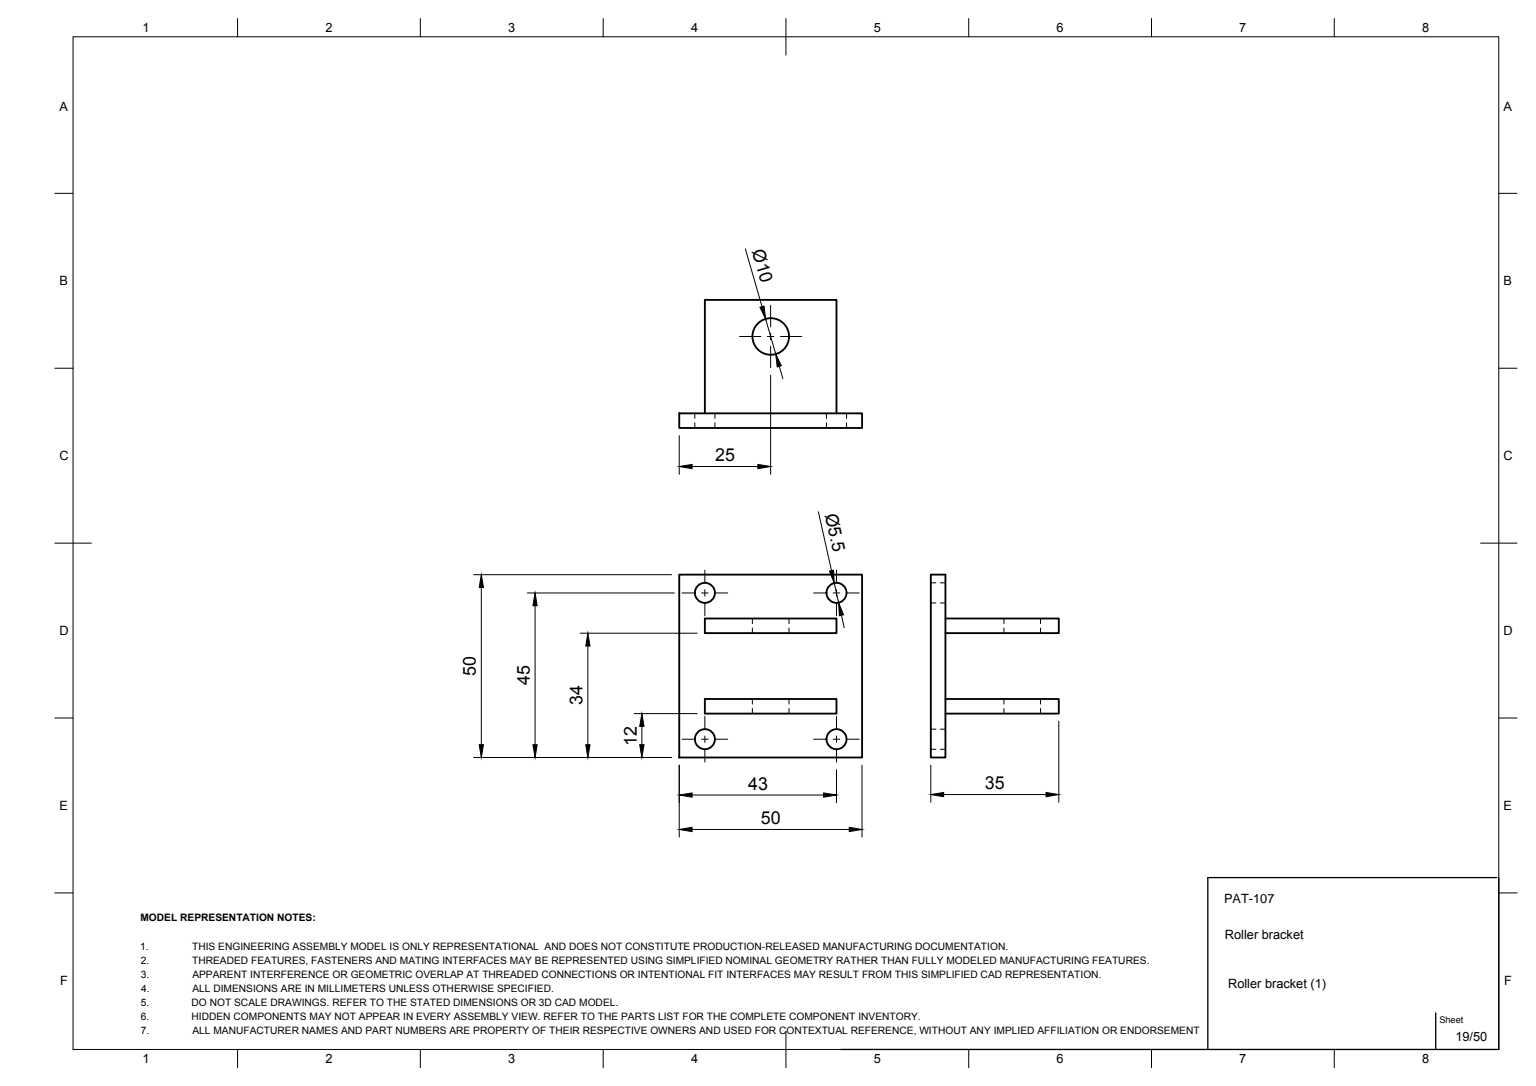
ISO-10303-21;
HEADER;
/* Generated by software containing ST-Developer
 * from STEP Tools, Inc. (www.steptools.com) 
 */

FILE_DESCRIPTION(
/* description */ ('Turntable on roller ring'),
/* implementation_level */ '2;1');

FILE_NAME(
/* name */ 'Roller bracket.step',
/* time_stamp */ '2026-10-28T03:23:59-07:00',
/* author */ (''),
/* organization */ (''),
/* preprocessor_version */ 'ST-DEVELOPER v20.2',
/* originating_system */ 'Autodesk Translation Framework v15.17.0.0',
/* authorisation */ '');

FILE_SCHEMA (('AUTOMOTIVE_DESIGN { 1 0 10303 214 3 1 1 }'));
ENDSEC;

DATA;
#10=MECHANICAL_DESIGN_GEOMETRIC_PRESENTATION_REPRESENTATION('',(#642),#16281);
#523=SHAPE_REPRESENTATION_RELATIONSHIP('SRR','None',#16540,#578);
#578=ADVANCED_BREP_SHAPE_REPRESENTATION('',(#712),#16234);
#642=STYLED_ITEM('',(#16911),#712);
#712=MANIFOLD_SOLID_BREP('Body1',#8385);
#867=FACE_BOUND('',#2085,.T.);
#868=FACE_BOUND('',#2087,.T.);
#869=FACE_BOUND('',#2092,.T.);
#870=FACE_BOUND('',#2094,.T.);
#871=FACE_BOUND('',#2100,.T.);
#872=FACE_BOUND('',#2101,.T.);
#873=FACE_BOUND('',#2102,.T.);
#874=FACE_BOUND('',#2103,.T.);
#875=FACE_BOUND('',#2104,.T.);
#876=FACE_BOUND('',#2105,.T.);
#877=FACE_BOUND('',#2107,.T.);
#878=FACE_BOUND('',#2108,.T.);
#879=FACE_BOUND('',#2109,.T.);
#880=FACE_BOUND('',#2110,.T.);
#1083=PLANE('',#9552);
#1084=PLANE('',#9553);
#1085=PLANE('',#9554);
#1086=PLANE('',#9555);
#1087=PLANE('',#9556);
#1088=PLANE('',#9557);
#1089=PLANE('',#9558);
#1090=PLANE('',#9559);
#1091=PLANE('',#9560);
#1092=PLANE('',#9561);
#1093=PLANE('',#9562);
#1094=PLANE('',#9563);
#1095=PLANE('',#9564);
#1096=PLANE('',#9565);
#1097=PLANE('',#9566);
#1098=PLANE('',#9567);
#1460=FACE_OUTER_BOUND('',#2075,.T.);
#1461=FACE_OUTER_BOUND('',#2076,.T.);
#1462=FACE_OUTER_BOUND('',#2077,.T.);
#1463=FACE_OUTER_BOUND('',#2078,.T.);
#1464=FACE_OUTER_BOUND('',#2079,.T.);
#1465=FACE_OUTER_BOUND('',#2080,.T.);
#1466=FACE_OUTER_BOUND('',#2081,.T.);
#1467=FACE_OUTER_BOUND('',#2082,.T.);
#1468=FACE_OUTER_BOUND('',#2083,.T.);
#1469=FACE_OUTER_BOUND('',#2084,.T.);
#1470=FACE_OUTER_BOUND('',#2086,.T.);
#1471=FACE_OUTER_BOUND('',#2088,.T.);
#1472=FACE_OUTER_BOUND('',#2089,.T.);
#1473=FACE_OUTER_BOUND('',#2090,.T.);
#1474=FACE_OUTER_BOUND('',#2091,.T.);
#1475=FACE_OUTER_BOUND('',#2093,.T.);
#1476=FACE_OUTER_BOUND('',#2095,.T.);
#1477=FACE_OUTER_BOUND('',#2096,.T.);
#1478=FACE_OUTER_BOUND('',#2097,.T.);
#1479=FACE_OUTER_BOUND('',#2098,.T.);
#1480=FACE_OUTER_BOUND('',#2099,.T.);
#1481=FACE_OUTER_BOUND('',#2106,.T.);
#2075=EDGE_LOOP('',(#6545,#6546,#6547,#6548));
#2076=EDGE_LOOP('',(#6549,#6550,#6551,#6552));
#2077=EDGE_LOOP('',(#6553,#6554,#6555,#6556));
#2078=EDGE_LOOP('',(#6557,#6558,#6559,#6560));
#2079=EDGE_LOOP('',(#6561,#6562,#6563,#6564));
#2080=EDGE_LOOP('',(#6565,#6566,#6567,#6568));
#2081=EDGE_LOOP('',(#6569,#6570,#6571,#6572));
#2082=EDGE_LOOP('',(#6573,#6574,#6575,#6576));
#2083=EDGE_LOOP('',(#6577,#6578,#6579,#6580));
#2084=EDGE_LOOP('',(#6581,#6582,#6583,#6584));
#2085=EDGE_LOOP('',(#6585));
#2086=EDGE_LOOP('',(#6586,#6587,#6588,#6589));
#2087=EDGE_LOOP('',(#6590));
#2088=EDGE_LOOP('',(#6591,#6592,#6593,#6594));
#2089=EDGE_LOOP('',(#6595,#6596,#6597,#6598));
#2090=EDGE_LOOP('',(#6599,#6600,#6601,#6602));
#2091=EDGE_LOOP('',(#6603,#6604,#6605,#6606));
#2092=EDGE_LOOP('',(#6607));
#2093=EDGE_LOOP('',(#6608,#6609,#6610,#6611));
#2094=EDGE_LOOP('',(#6612));
#2095=EDGE_LOOP('',(#6613,#6614,#6615,#6616));
#2096=EDGE_LOOP('',(#6617,#6618,#6619,#6620));
#2097=EDGE_LOOP('',(#6621,#6622,#6623,#6624));
#2098=EDGE_LOOP('',(#6625,#6626,#6627,#6628));
#2099=EDGE_LOOP('',(#6629,#6630,#6631,#6632));
#2100=EDGE_LOOP('',(#6633,#6634,#6635,#6636));
#2101=EDGE_LOOP('',(#6637,#6638,#6639,#6640));
#2102=EDGE_LOOP('',(#6641));
#2103=EDGE_LOOP('',(#6642));
#2104=EDGE_LOOP('',(#6643));
#2105=EDGE_LOOP('',(#6644));
#2106=EDGE_LOOP('',(#6645,#6646,#6647,#6648));
#2107=EDGE_LOOP('',(#6649));
#2108=EDGE_LOOP('',(#6650));
#2109=EDGE_LOOP('',(#6651));
#2110=EDGE_LOOP('',(#6652));
#2686=LINE('',#14454,#3169);
#2687=LINE('',#14460,#3170);
#2688=LINE('',#14466,#3171);
#2689=LINE('',#14472,#3172);
#2690=LINE('',#14478,#3173);
#2691=LINE('',#14484,#3174);
#2692=LINE('',#14489,#3175);
#2693=LINE('',#14491,#3176);
#2694=LINE('',#14493,#3177);
#2695=LINE('',#14494,#3178);
#2696=LINE('',#14498,#3179);
#2697=LINE('',#14500,#3180);
#2698=LINE('',#14502,#3181);
#2699=LINE('',#14503,#3182);
#2700=LINE('',#14505,#3183);
#2701=LINE('',#14506,#3184);
#2702=LINE('',#14508,#3185);
#2703=LINE('',#14510,#3186);
#2704=LINE('',#14514,#3187);
#2705=LINE('',#14516,#3188);
#2706=LINE('',#14518,#3189);
#2707=LINE('',#14519,#3190);
#2708=LINE('',#14523,#3191);
#2709=LINE('',#14525,#3192);
#2710=LINE('',#14527,#3193);
#2711=LINE('',#14528,#3194);
#2712=LINE('',#14530,#3195);
#2713=LINE('',#14531,#3196);
#2714=LINE('',#14533,#3197);
#2715=LINE('',#14535,#3198);
#2716=LINE('',#14539,#3199);
#2717=LINE('',#14541,#3200);
#2718=LINE('',#14543,#3201);
#2719=LINE('',#14544,#3202);
#2720=LINE('',#14547,#3203);
#2721=LINE('',#14549,#3204);
#2722=LINE('',#14550,#3205);
#2723=LINE('',#14553,#3206);
#2724=LINE('',#14555,#3207);
#2725=LINE('',#14556,#3208);
#2726=LINE('',#14558,#3209);
#2727=LINE('',#14559,#3210);
#3169=VECTOR('',#11385,0.275);
#3170=VECTOR('',#11392,0.275);
#3171=VECTOR('',#11399,0.275);
#3172=VECTOR('',#11406,0.275);
#3173=VECTOR('',#11413,0.5);
#3174=VECTOR('',#11420,0.5);
#3175=VECTOR('',#11425,1.);
#3176=VECTOR('',#11426,1.);
#3177=VECTOR('',#11427,1.);
#3178=VECTOR('',#11428,1.);
#3179=VECTOR('',#11431,1.);
#3180=VECTOR('',#11432,1.);
#3181=VECTOR('',#11433,1.);
#3182=VECTOR('',#11434,1.);
#3183=VECTOR('',#11437,1.);
#3184=VECTOR('',#11438,1.);
#3185=VECTOR('',#11441,1.);
#3186=VECTOR('',#11444,1.);
#3187=VECTOR('',#11447,1.);
#3188=VECTOR('',#11448,1.);
#3189=VECTOR('',#11449,1.);
#3190=VECTOR('',#11450,1.);
#3191=VECTOR('',#11453,1.);
#3192=VECTOR('',#11454,1.);
#3193=VECTOR('',#11455,1.);
#3194=VECTOR('',#11456,1.);
#3195=VECTOR('',#11459,1.);
#3196=VECTOR('',#11460,1.);
#3197=VECTOR('',#11463,1.);
#3198=VECTOR('',#11466,1.);
#3199=VECTOR('',#11469,1.);
#3200=VECTOR('',#11470,1.);
#3201=VECTOR('',#11471,1.);
#3202=VECTOR('',#11472,1.);
#3203=VECTOR('',#11475,1.);
#3204=VECTOR('',#11476,1.);
#3205=VECTOR('',#11477,1.);
#3206=VECTOR('',#11480,1.);
#3207=VECTOR('',#11481,1.);
#3208=VECTOR('',#11482,1.);
#3209=VECTOR('',#11485,1.);
#3210=VECTOR('',#11486,1.);
#3695=CIRCLE('',#9535,0.275);
#3696=CIRCLE('',#9536,0.275);
#3697=CIRCLE('',#9538,0.275);
#3698=CIRCLE('',#9539,0.275);
#3699=CIRCLE('',#9541,0.275);
#3700=CIRCLE('',#9542,0.275);
#3701=CIRCLE('',#9544,0.275);
#3702=CIRCLE('',#9545,0.275);
#3703=CIRCLE('',#9547,0.5);
#3704=CIRCLE('',#9548,0.5);
#3705=CIRCLE('',#9550,0.5);
#3706=CIRCLE('',#9551,0.5);
#4251=VERTEX_POINT('',#14451);
#4252=VERTEX_POINT('',#14453);
#4253=VERTEX_POINT('',#14457);
#4254=VERTEX_POINT('',#14459);
#4255=VERTEX_POINT('',#14463);
#4256=VERTEX_POINT('',#14465);
#4257=VERTEX_POINT('',#14469);
#4258=VERTEX_POINT('',#14471);
#4259=VERTEX_POINT('',#14475);
#4260=VERTEX_POINT('',#14477);
#4261=VERTEX_POINT('',#14481);
#4262=VERTEX_POINT('',#14483);
#4263=VERTEX_POINT('',#14487);
#4264=VERTEX_POINT('',#14488);
#4265=VERTEX_POINT('',#14490);
#4266=VERTEX_POINT('',#14492);
#4267=VERTEX_POINT('',#14496);
#4268=VERTEX_POINT('',#14497);
#4269=VERTEX_POINT('',#14499);
#4270=VERTEX_POINT('',#14501);
#4271=VERTEX_POINT('',#14512);
#4272=VERTEX_POINT('',#14513);
#4273=VERTEX_POINT('',#14515);
#4274=VERTEX_POINT('',#14517);
#4275=VERTEX_POINT('',#14521);
#4276=VERTEX_POINT('',#14522);
#4277=VERTEX_POINT('',#14524);
#4278=VERTEX_POINT('',#14526);
#4279=VERTEX_POINT('',#14537);
#4280=VERTEX_POINT('',#14538);
#4281=VERTEX_POINT('',#14540);
#4282=VERTEX_POINT('',#14542);
#4283=VERTEX_POINT('',#14546);
#4284=VERTEX_POINT('',#14548);
#4285=VERTEX_POINT('',#14552);
#4286=VERTEX_POINT('',#14554);
#5083=EDGE_CURVE('',#4251,#4251,#3695,.T.);
#5084=EDGE_CURVE('',#4251,#4252,#2686,.T.);
#5085=EDGE_CURVE('',#4252,#4252,#3696,.T.);
#5086=EDGE_CURVE('',#4253,#4253,#3697,.T.);
#5087=EDGE_CURVE('',#4253,#4254,#2687,.T.);
#5088=EDGE_CURVE('',#4254,#4254,#3698,.T.);
#5089=EDGE_CURVE('',#4255,#4255,#3699,.T.);
#5090=EDGE_CURVE('',#4255,#4256,#2688,.T.);
#5091=EDGE_CURVE('',#4256,#4256,#3700,.T.);
#5092=EDGE_CURVE('',#4257,#4257,#3701,.T.);
#5093=EDGE_CURVE('',#4257,#4258,#2689,.T.);
#5094=EDGE_CURVE('',#4258,#4258,#3702,.T.);
#5095=EDGE_CURVE('',#4259,#4259,#3703,.T.);
#5096=EDGE_CURVE('',#4259,#4260,#2690,.T.);
#5097=EDGE_CURVE('',#4260,#4260,#3704,.T.);
#5098=EDGE_CURVE('',#4261,#4261,#3705,.T.);
#5099=EDGE_CURVE('',#4261,#4262,#2691,.T.);
#5100=EDGE_CURVE('',#4262,#4262,#3706,.T.);
#5101=EDGE_CURVE('',#4263,#4264,#2692,.T.);
#5102=EDGE_CURVE('',#4263,#4265,#2693,.T.);
#5103=EDGE_CURVE('',#4266,#4265,#2694,.T.);
#5104=EDGE_CURVE('',#4264,#4266,#2695,.T.);
#5105=EDGE_CURVE('',#4267,#4268,#2696,.T.);
#5106=EDGE_CURVE('',#4269,#4267,#2697,.T.);
#5107=EDGE_CURVE('',#4270,#4269,#2698,.T.);
#5108=EDGE_CURVE('',#4268,#4270,#2699,.T.);
#5109=EDGE_CURVE('',#4268,#4263,#2700,.T.);
#5110=EDGE_CURVE('',#4265,#4270,#2701,.T.);
#5111=EDGE_CURVE('',#4266,#4269,#2702,.T.);
#5112=EDGE_CURVE('',#4267,#4264,#2703,.T.);
#5113=EDGE_CURVE('',#4271,#4272,#2704,.T.);
#5114=EDGE_CURVE('',#4271,#4273,#2705,.T.);
#5115=EDGE_CURVE('',#4274,#4273,#2706,.T.);
#5116=EDGE_CURVE('',#4272,#4274,#2707,.T.);
#5117=EDGE_CURVE('',#4275,#4276,#2708,.T.);
#5118=EDGE_CURVE('',#4277,#4275,#2709,.T.);
#5119=EDGE_CURVE('',#4278,#4277,#2710,.T.);
#5120=EDGE_CURVE('',#4276,#4278,#2711,.T.);
#5121=EDGE_CURVE('',#4276,#4271,#2712,.T.);
#5122=EDGE_CURVE('',#4273,#4278,#2713,.T.);
#5123=EDGE_CURVE('',#4274,#4277,#2714,.T.);
#5124=EDGE_CURVE('',#4275,#4272,#2715,.T.);
#5125=EDGE_CURVE('',#4279,#4280,#2716,.T.);
#5126=EDGE_CURVE('',#4280,#4281,#2717,.T.);
#5127=EDGE_CURVE('',#4282,#4281,#2718,.T.);
#5128=EDGE_CURVE('',#4279,#4282,#2719,.T.);
#5129=EDGE_CURVE('',#4283,#4279,#2720,.T.);
#5130=EDGE_CURVE('',#4284,#4282,#2721,.T.);
#5131=EDGE_CURVE('',#4283,#4284,#2722,.T.);
#5132=EDGE_CURVE('',#4285,#4283,#2723,.T.);
#5133=EDGE_CURVE('',#4286,#4284,#2724,.T.);
#5134=EDGE_CURVE('',#4285,#4286,#2725,.T.);
#5135=EDGE_CURVE('',#4280,#4285,#2726,.T.);
#5136=EDGE_CURVE('',#4281,#4286,#2727,.T.);
#6545=ORIENTED_EDGE('',*,*,#5083,.F.);
#6546=ORIENTED_EDGE('',*,*,#5084,.T.);
#6547=ORIENTED_EDGE('',*,*,#5085,.F.);
#6548=ORIENTED_EDGE('',*,*,#5084,.F.);
#6549=ORIENTED_EDGE('',*,*,#5086,.F.);
#6550=ORIENTED_EDGE('',*,*,#5087,.T.);
#6551=ORIENTED_EDGE('',*,*,#5088,.F.);
#6552=ORIENTED_EDGE('',*,*,#5087,.F.);
#6553=ORIENTED_EDGE('',*,*,#5089,.F.);
#6554=ORIENTED_EDGE('',*,*,#5090,.T.);
#6555=ORIENTED_EDGE('',*,*,#5091,.F.);
#6556=ORIENTED_EDGE('',*,*,#5090,.F.);
#6557=ORIENTED_EDGE('',*,*,#5092,.F.);
#6558=ORIENTED_EDGE('',*,*,#5093,.T.);
#6559=ORIENTED_EDGE('',*,*,#5094,.F.);
#6560=ORIENTED_EDGE('',*,*,#5093,.F.);
#6561=ORIENTED_EDGE('',*,*,#5095,.F.);
#6562=ORIENTED_EDGE('',*,*,#5096,.T.);
#6563=ORIENTED_EDGE('',*,*,#5097,.F.);
#6564=ORIENTED_EDGE('',*,*,#5096,.F.);
#6565=ORIENTED_EDGE('',*,*,#5098,.F.);
#6566=ORIENTED_EDGE('',*,*,#5099,.T.);
#6567=ORIENTED_EDGE('',*,*,#5100,.F.);
#6568=ORIENTED_EDGE('',*,*,#5099,.F.);
#6569=ORIENTED_EDGE('',*,*,#5101,.F.);
#6570=ORIENTED_EDGE('',*,*,#5102,.T.);
#6571=ORIENTED_EDGE('',*,*,#5103,.F.);
#6572=ORIENTED_EDGE('',*,*,#5104,.F.);
#6573=ORIENTED_EDGE('',*,*,#5105,.F.);
#6574=ORIENTED_EDGE('',*,*,#5106,.F.);
#6575=ORIENTED_EDGE('',*,*,#5107,.F.);
#6576=ORIENTED_EDGE('',*,*,#5108,.F.);
#6577=ORIENTED_EDGE('',*,*,#5109,.F.);
#6578=ORIENTED_EDGE('',*,*,#5108,.T.);
#6579=ORIENTED_EDGE('',*,*,#5110,.F.);
#6580=ORIENTED_EDGE('',*,*,#5102,.F.);
#6581=ORIENTED_EDGE('',*,*,#5110,.T.);
#6582=ORIENTED_EDGE('',*,*,#5107,.T.);
#6583=ORIENTED_EDGE('',*,*,#5111,.F.);
#6584=ORIENTED_EDGE('',*,*,#5103,.T.);
#6585=ORIENTED_EDGE('',*,*,#5100,.T.);
#6586=ORIENTED_EDGE('',*,*,#5109,.T.);
#6587=ORIENTED_EDGE('',*,*,#5101,.T.);
#6588=ORIENTED_EDGE('',*,*,#5112,.F.);
#6589=ORIENTED_EDGE('',*,*,#5105,.T.);
#6590=ORIENTED_EDGE('',*,*,#5098,.T.);
#6591=ORIENTED_EDGE('',*,*,#5113,.F.);
#6592=ORIENTED_EDGE('',*,*,#5114,.T.);
#6593=ORIENTED_EDGE('',*,*,#5115,.F.);
#6594=ORIENTED_EDGE('',*,*,#5116,.F.);
#6595=ORIENTED_EDGE('',*,*,#5117,.F.);
#6596=ORIENTED_EDGE('',*,*,#5118,.F.);
#6597=ORIENTED_EDGE('',*,*,#5119,.F.);
#6598=ORIENTED_EDGE('',*,*,#5120,.F.);
#6599=ORIENTED_EDGE('',*,*,#5121,.F.);
#6600=ORIENTED_EDGE('',*,*,#5120,.T.);
#6601=ORIENTED_EDGE('',*,*,#5122,.F.);
#6602=ORIENTED_EDGE('',*,*,#5114,.F.);
#6603=ORIENTED_EDGE('',*,*,#5122,.T.);
#6604=ORIENTED_EDGE('',*,*,#5119,.T.);
#6605=ORIENTED_EDGE('',*,*,#5123,.F.);
#6606=ORIENTED_EDGE('',*,*,#5115,.T.);
#6607=ORIENTED_EDGE('',*,*,#5097,.T.);
#6608=ORIENTED_EDGE('',*,*,#5121,.T.);
#6609=ORIENTED_EDGE('',*,*,#5113,.T.);
#6610=ORIENTED_EDGE('',*,*,#5124,.F.);
#6611=ORIENTED_EDGE('',*,*,#5117,.T.);
#6612=ORIENTED_EDGE('',*,*,#5095,.T.);
#6613=ORIENTED_EDGE('',*,*,#5125,.T.);
#6614=ORIENTED_EDGE('',*,*,#5126,.T.);
#6615=ORIENTED_EDGE('',*,*,#5127,.F.);
#6616=ORIENTED_EDGE('',*,*,#5128,.F.);
#6617=ORIENTED_EDGE('',*,*,#5129,.T.);
#6618=ORIENTED_EDGE('',*,*,#5128,.T.);
#6619=ORIENTED_EDGE('',*,*,#5130,.F.);
#6620=ORIENTED_EDGE('',*,*,#5131,.F.);
#6621=ORIENTED_EDGE('',*,*,#5132,.T.);
#6622=ORIENTED_EDGE('',*,*,#5131,.T.);
#6623=ORIENTED_EDGE('',*,*,#5133,.F.);
#6624=ORIENTED_EDGE('',*,*,#5134,.F.);
#6625=ORIENTED_EDGE('',*,*,#5135,.T.);
#6626=ORIENTED_EDGE('',*,*,#5134,.T.);
#6627=ORIENTED_EDGE('',*,*,#5136,.F.);
#6628=ORIENTED_EDGE('',*,*,#5126,.F.);
#6629=ORIENTED_EDGE('',*,*,#5136,.T.);
#6630=ORIENTED_EDGE('',*,*,#5133,.T.);
#6631=ORIENTED_EDGE('',*,*,#5130,.T.);
#6632=ORIENTED_EDGE('',*,*,#5127,.T.);
#6633=ORIENTED_EDGE('',*,*,#5118,.T.);
#6634=ORIENTED_EDGE('',*,*,#5124,.T.);
#6635=ORIENTED_EDGE('',*,*,#5116,.T.);
#6636=ORIENTED_EDGE('',*,*,#5123,.T.);
#6637=ORIENTED_EDGE('',*,*,#5106,.T.);
#6638=ORIENTED_EDGE('',*,*,#5112,.T.);
#6639=ORIENTED_EDGE('',*,*,#5104,.T.);
#6640=ORIENTED_EDGE('',*,*,#5111,.T.);
#6641=ORIENTED_EDGE('',*,*,#5094,.T.);
#6642=ORIENTED_EDGE('',*,*,#5091,.T.);
#6643=ORIENTED_EDGE('',*,*,#5088,.T.);
#6644=ORIENTED_EDGE('',*,*,#5085,.T.);
#6645=ORIENTED_EDGE('',*,*,#5135,.F.);
#6646=ORIENTED_EDGE('',*,*,#5125,.F.);
#6647=ORIENTED_EDGE('',*,*,#5129,.F.);
#6648=ORIENTED_EDGE('',*,*,#5132,.F.);
#6649=ORIENTED_EDGE('',*,*,#5083,.T.);
#6650=ORIENTED_EDGE('',*,*,#5086,.T.);
#6651=ORIENTED_EDGE('',*,*,#5089,.T.);
#6652=ORIENTED_EDGE('',*,*,#5092,.T.);
#7753=CYLINDRICAL_SURFACE('',#9534,0.275);
#7754=CYLINDRICAL_SURFACE('',#9537,0.275);
#7755=CYLINDRICAL_SURFACE('',#9540,0.275);
#7756=CYLINDRICAL_SURFACE('',#9543,0.275);
#7757=CYLINDRICAL_SURFACE('',#9546,0.5);
#7758=CYLINDRICAL_SURFACE('',#9549,0.5);
#8063=ADVANCED_FACE('',(#1460),#7753,.F.);
#8064=ADVANCED_FACE('',(#1461),#7754,.F.);
#8065=ADVANCED_FACE('',(#1462),#7755,.F.);
#8066=ADVANCED_FACE('',(#1463),#7756,.F.);
#8067=ADVANCED_FACE('',(#1464),#7757,.F.);
#8068=ADVANCED_FACE('',(#1465),#7758,.F.);
#8069=ADVANCED_FACE('',(#1466),#1083,.T.);
#8070=ADVANCED_FACE('',(#1467),#1084,.T.);
#8071=ADVANCED_FACE('',(#1468),#1085,.T.);
#8072=ADVANCED_FACE('',(#1469,#867),#1086,.T.);
#8073=ADVANCED_FACE('',(#1470,#868),#1087,.F.);
#8074=ADVANCED_FACE('',(#1471),#1088,.T.);
#8075=ADVANCED_FACE('',(#1472),#1089,.T.);
#8076=ADVANCED_FACE('',(#1473),#1090,.T.);
#8077=ADVANCED_FACE('',(#1474,#869),#1091,.T.);
#8078=ADVANCED_FACE('',(#1475,#870),#1092,.F.);
#8079=ADVANCED_FACE('',(#1476),#1093,.T.);
#8080=ADVANCED_FACE('',(#1477),#1094,.T.);
#8081=ADVANCED_FACE('',(#1478),#1095,.T.);
#8082=ADVANCED_FACE('',(#1479),#1096,.T.);
#8083=ADVANCED_FACE('',(#1480,#871,#872,#873,#874,#875,#876),#1097,.T.);
#8084=ADVANCED_FACE('',(#1481,#877,#878,#879,#880),#1098,.F.);
#8385=CLOSED_SHELL('',(#8063,#8064,#8065,#8066,#8067,#8068,#8069,#8070,
#8071,#8072,#8073,#8074,#8075,#8076,#8077,#8078,#8079,#8080,#8081,#8082,
#8083,#8084));
#9533=AXIS2_PLACEMENT_3D('',#14449,#11379,#11380);
#9534=AXIS2_PLACEMENT_3D('',#14450,#11381,#11382);
#9535=AXIS2_PLACEMENT_3D('',#14452,#11383,#11384);
#9536=AXIS2_PLACEMENT_3D('',#14455,#11386,#11387);
#9537=AXIS2_PLACEMENT_3D('',#14456,#11388,#11389);
#9538=AXIS2_PLACEMENT_3D('',#14458,#11390,#11391);
#9539=AXIS2_PLACEMENT_3D('',#14461,#11393,#11394);
#9540=AXIS2_PLACEMENT_3D('',#14462,#11395,#11396);
#9541=AXIS2_PLACEMENT_3D('',#14464,#11397,#11398);
#9542=AXIS2_PLACEMENT_3D('',#14467,#11400,#11401);
#9543=AXIS2_PLACEMENT_3D('',#14468,#11402,#11403);
#9544=AXIS2_PLACEMENT_3D('',#14470,#11404,#11405);
#9545=AXIS2_PLACEMENT_3D('',#14473,#11407,#11408);
#9546=AXIS2_PLACEMENT_3D('',#14474,#11409,#11410);
#9547=AXIS2_PLACEMENT_3D('',#14476,#11411,#11412);
#9548=AXIS2_PLACEMENT_3D('',#14479,#11414,#11415);
#9549=AXIS2_PLACEMENT_3D('',#14480,#11416,#11417);
#9550=AXIS2_PLACEMENT_3D('',#14482,#11418,#11419);
#9551=AXIS2_PLACEMENT_3D('',#14485,#11421,#11422);
#9552=AXIS2_PLACEMENT_3D('',#14486,#11423,#11424);
#9553=AXIS2_PLACEMENT_3D('',#14495,#11429,#11430);
#9554=AXIS2_PLACEMENT_3D('',#14504,#11435,#11436);
#9555=AXIS2_PLACEMENT_3D('',#14507,#11439,#11440);
#9556=AXIS2_PLACEMENT_3D('',#14509,#11442,#11443);
#9557=AXIS2_PLACEMENT_3D('',#14511,#11445,#11446);
#9558=AXIS2_PLACEMENT_3D('',#14520,#11451,#11452);
#9559=AXIS2_PLACEMENT_3D('',#14529,#11457,#11458);
#9560=AXIS2_PLACEMENT_3D('',#14532,#11461,#11462);
#9561=AXIS2_PLACEMENT_3D('',#14534,#11464,#11465);
#9562=AXIS2_PLACEMENT_3D('',#14536,#11467,#11468);
#9563=AXIS2_PLACEMENT_3D('',#14545,#11473,#11474);
#9564=AXIS2_PLACEMENT_3D('',#14551,#11478,#11479);
#9565=AXIS2_PLACEMENT_3D('',#14557,#11483,#11484);
#9566=AXIS2_PLACEMENT_3D('',#14560,#11487,#11488);
#9567=AXIS2_PLACEMENT_3D('',#14561,#11489,#11490);
#11379=DIRECTION('axis',(0.,0.,1.));
#11380=DIRECTION('refdir',(1.,0.,0.));
#11381=DIRECTION('center_axis',(0.,0.,1.));
#11382=DIRECTION('ref_axis',(1.,0.,0.));
#11383=DIRECTION('center_axis',(0.,0.,1.));
#11384=DIRECTION('ref_axis',(1.,0.,0.));
#11385=DIRECTION('',(0.,0.,1.));
#11386=DIRECTION('center_axis',(0.,0.,-1.));
#11387=DIRECTION('ref_axis',(1.,0.,0.));
#11388=DIRECTION('center_axis',(0.,0.,1.));
#11389=DIRECTION('ref_axis',(1.,0.,0.));
#11390=DIRECTION('center_axis',(0.,0.,1.));
#11391=DIRECTION('ref_axis',(1.,0.,0.));
#11392=DIRECTION('',(0.,0.,1.));
#11393=DIRECTION('center_axis',(0.,0.,-1.));
#11394=DIRECTION('ref_axis',(1.,0.,0.));
#11395=DIRECTION('center_axis',(0.,0.,1.));
#11396=DIRECTION('ref_axis',(1.,0.,0.));
#11397=DIRECTION('center_axis',(0.,0.,1.));
#11398=DIRECTION('ref_axis',(1.,0.,0.));
#11399=DIRECTION('',(0.,0.,1.));
#11400=DIRECTION('center_axis',(0.,0.,-1.));
#11401=DIRECTION('ref_axis',(1.,0.,0.));
#11402=DIRECTION('center_axis',(0.,0.,1.));
#11403=DIRECTION('ref_axis',(1.,0.,0.));
#11404=DIRECTION('center_axis',(0.,0.,1.));
#11405=DIRECTION('ref_axis',(1.,0.,0.));
#11406=DIRECTION('',(0.,0.,1.));
#11407=DIRECTION('center_axis',(0.,0.,-1.));
#11408=DIRECTION('ref_axis',(1.,0.,0.));
#11409=DIRECTION('center_axis',(0.,1.,0.));
#11410=DIRECTION('ref_axis',(1.,0.,0.));
#11411=DIRECTION('center_axis',(0.,1.,0.));
#11412=DIRECTION('ref_axis',(1.,0.,0.));
#11413=DIRECTION('',(0.,1.,0.));
#11414=DIRECTION('center_axis',(0.,-1.,0.));
#11415=DIRECTION('ref_axis',(1.,0.,0.));
#11416=DIRECTION('center_axis',(0.,1.,0.));
#11417=DIRECTION('ref_axis',(1.,0.,0.));
#11418=DIRECTION('center_axis',(0.,1.,0.));
#11419=DIRECTION('ref_axis',(1.,0.,0.));
#11420=DIRECTION('',(0.,1.,0.));
#11421=DIRECTION('center_axis',(0.,-1.,0.));
#11422=DIRECTION('ref_axis',(1.,0.,0.));
#11423=DIRECTION('center_axis',(-1.,0.,0.));
#11424=DIRECTION('ref_axis',(0.,0.,1.));
#11425=DIRECTION('',(0.,0.,-1.));
#11426=DIRECTION('',(0.,1.,0.));
#11427=DIRECTION('',(0.,0.,1.));
#11428=DIRECTION('',(0.,1.,0.));
#11429=DIRECTION('center_axis',(1.,0.,0.));
#11430=DIRECTION('ref_axis',(0.,0.,-1.));
#11431=DIRECTION('',(0.,0.,1.));
#11432=DIRECTION('',(0.,-1.,0.));
#11433=DIRECTION('',(0.,0.,-1.));
#11434=DIRECTION('',(0.,1.,0.));
#11435=DIRECTION('center_axis',(0.,0.,1.));
#11436=DIRECTION('ref_axis',(1.,0.,0.));
#11437=DIRECTION('',(-1.,0.,0.));
#11438=DIRECTION('',(1.,0.,0.));
#11439=DIRECTION('center_axis',(0.,1.,0.));
#11440=DIRECTION('ref_axis',(0.,0.,1.));
#11441=DIRECTION('',(1.,0.,0.));
#11442=DIRECTION('center_axis',(0.,1.,0.));
#11443=DIRECTION('ref_axis',(1.,0.,0.));
#11444=DIRECTION('',(-1.,0.,0.));
#11445=DIRECTION('center_axis',(-1.,0.,0.));
#11446=DIRECTION('ref_axis',(0.,0.,1.));
#11447=DIRECTION('',(0.,0.,-1.));
#11448=DIRECTION('',(0.,1.,0.));
#11449=DIRECTION('',(0.,0.,1.));
#11450=DIRECTION('',(0.,1.,0.));
#11451=DIRECTION('center_axis',(1.,0.,0.));
#11452=DIRECTION('ref_axis',(0.,0.,-1.));
#11453=DIRECTION('',(0.,0.,1.));
#11454=DIRECTION('',(0.,-1.,0.));
#11455=DIRECTION('',(0.,0.,-1.));
#11456=DIRECTION('',(0.,1.,0.));
#11457=DIRECTION('center_axis',(0.,0.,1.));
#11458=DIRECTION('ref_axis',(1.,0.,0.));
#11459=DIRECTION('',(-1.,0.,0.));
#11460=DIRECTION('',(1.,0.,0.));
#11461=DIRECTION('center_axis',(0.,1.,0.));
#11462=DIRECTION('ref_axis',(0.,0.,1.));
#11463=DIRECTION('',(1.,0.,0.));
#11464=DIRECTION('center_axis',(0.,1.,0.));
#11465=DIRECTION('ref_axis',(1.,0.,0.));
#11466=DIRECTION('',(-1.,0.,0.));
#11467=DIRECTION('center_axis',(0.,1.,0.));
#11468=DIRECTION('ref_axis',(-1.,0.,0.));
#11469=DIRECTION('',(-1.,0.,0.));
#11470=DIRECTION('',(0.,0.,1.));
#11471=DIRECTION('',(-1.,0.,0.));
#11472=DIRECTION('',(0.,0.,1.));
#11473=DIRECTION('center_axis',(1.,0.,0.));
#11474=DIRECTION('ref_axis',(0.,1.,0.));
#11475=DIRECTION('',(0.,1.,0.));
#11476=DIRECTION('',(0.,1.,0.));
#11477=DIRECTION('',(0.,0.,1.));
#11478=DIRECTION('center_axis',(0.,-1.,0.));
#11479=DIRECTION('ref_axis',(1.,0.,0.));
#11480=DIRECTION('',(1.,0.,0.));
#11481=DIRECTION('',(1.,0.,0.));
#11482=DIRECTION('',(0.,0.,1.));
#11483=DIRECTION('center_axis',(-1.,0.,0.));
#11484=DIRECTION('ref_axis',(0.,-1.,0.));
#11485=DIRECTION('',(0.,-1.,0.));
#11486=DIRECTION('',(0.,-1.,0.));
#11487=DIRECTION('center_axis',(0.,0.,1.));
#11488=DIRECTION('ref_axis',(1.,0.,0.));
#11489=DIRECTION('center_axis',(0.,0.,1.));
#11490=DIRECTION('ref_axis',(1.,0.,0.));
#14449=CARTESIAN_POINT('',(0.,0.,0.));
#14450=CARTESIAN_POINT('Origin',(1.8,13.,0.9));
#14451=CARTESIAN_POINT('',(1.525,13.,1.));
#14452=CARTESIAN_POINT('Origin',(1.8,13.,1.));
#14453=CARTESIAN_POINT('',(1.525,13.,1.4));
#14454=CARTESIAN_POINT('',(1.525,13.,0.9));
#14455=CARTESIAN_POINT('Origin',(1.8,13.,1.4));
#14456=CARTESIAN_POINT('Origin',(-1.8,17.,0.9));
#14457=CARTESIAN_POINT('',(-2.075,17.,1.));
#14458=CARTESIAN_POINT('Origin',(-1.8,17.,1.));
#14459=CARTESIAN_POINT('',(-2.075,17.,1.4));
#14460=CARTESIAN_POINT('',(-2.075,17.,0.9));
#14461=CARTESIAN_POINT('Origin',(-1.8,17.,1.4));
#14462=CARTESIAN_POINT('Origin',(-1.8,13.,0.9));
#14463=CARTESIAN_POINT('',(-2.075,13.,1.));
#14464=CARTESIAN_POINT('Origin',(-1.8,13.,1.));
#14465=CARTESIAN_POINT('',(-2.075,13.,1.4));
#14466=CARTESIAN_POINT('',(-2.075,13.,0.9));
#14467=CARTESIAN_POINT('Origin',(-1.8,13.,1.4));
#14468=CARTESIAN_POINT('Origin',(1.8,17.,0.9));
#14469=CARTESIAN_POINT('',(1.525,17.,1.));
#14470=CARTESIAN_POINT('Origin',(1.8,17.,1.));
#14471=CARTESIAN_POINT('',(1.525,17.,1.4));
#14472=CARTESIAN_POINT('',(1.525,17.,0.9));
#14473=CARTESIAN_POINT('Origin',(1.8,17.,1.4));
#14474=CARTESIAN_POINT('Origin',(0.,13.6,3.5));
#14475=CARTESIAN_POINT('',(-0.5,13.7,3.5));
#14476=CARTESIAN_POINT('Origin',(0.,13.7,3.5));
#14477=CARTESIAN_POINT('',(-0.5,14.1,3.5));
#14478=CARTESIAN_POINT('',(-0.5,13.6,3.5));
#14479=CARTESIAN_POINT('Origin',(0.,14.1,3.5));
#14480=CARTESIAN_POINT('Origin',(0.,13.6,3.5));
#14481=CARTESIAN_POINT('',(-0.5,15.9,3.5));
#14482=CARTESIAN_POINT('Origin',(0.,15.9,3.5));
#14483=CARTESIAN_POINT('',(-0.5,16.3,3.5));
#14484=CARTESIAN_POINT('',(-0.5,13.6,3.5));
#14485=CARTESIAN_POINT('Origin',(0.,16.3,3.5));
#14486=CARTESIAN_POINT('Origin',(-1.8,15.9,1.4));
#14487=CARTESIAN_POINT('',(-1.8,15.9,4.5));
#14488=CARTESIAN_POINT('',(-1.8,15.9,1.4));
#14489=CARTESIAN_POINT('',(-1.8,15.9,4.5));
#14490=CARTESIAN_POINT('',(-1.8,16.3,4.5));
#14491=CARTESIAN_POINT('',(-1.8,15.9,4.5));
#14492=CARTESIAN_POINT('',(-1.8,16.3,1.4));
#14493=CARTESIAN_POINT('',(-1.8,16.3,4.5));
#14494=CARTESIAN_POINT('',(-1.8,15.45,1.4));
#14495=CARTESIAN_POINT('Origin',(1.8,15.9,4.5));
#14496=CARTESIAN_POINT('',(1.8,15.9,1.4));
#14497=CARTESIAN_POINT('',(1.8,15.9,4.5));
#14498=CARTESIAN_POINT('',(1.8,15.9,1.4));
#14499=CARTESIAN_POINT('',(1.8,16.3,1.4));
#14500=CARTESIAN_POINT('',(1.8,15.45,1.4));
#14501=CARTESIAN_POINT('',(1.8,16.3,4.5));
#14502=CARTESIAN_POINT('',(1.8,16.3,1.4));
#14503=CARTESIAN_POINT('',(1.8,15.9,4.5));
#14504=CARTESIAN_POINT('Origin',(-1.8,15.9,4.5));
#14505=CARTESIAN_POINT('',(1.8,15.9,4.5));
#14506=CARTESIAN_POINT('',(1.8,16.3,4.5));
#14507=CARTESIAN_POINT('Origin',(0.,16.3,2.95));
#14508=CARTESIAN_POINT('',(0.,16.3,1.4));
#14509=CARTESIAN_POINT('Origin',(0.,15.9,2.95));
#14510=CARTESIAN_POINT('',(0.,15.9,1.4));
#14511=CARTESIAN_POINT('Origin',(-1.8,13.7,1.4));
#14512=CARTESIAN_POINT('',(-1.8,13.7,4.5));
#14513=CARTESIAN_POINT('',(-1.8,13.7,1.4));
#14514=CARTESIAN_POINT('',(-1.8,13.7,4.5));
#14515=CARTESIAN_POINT('',(-1.8,14.1,4.5));
#14516=CARTESIAN_POINT('',(-1.8,13.7,4.5));
#14517=CARTESIAN_POINT('',(-1.8,14.1,1.4));
#14518=CARTESIAN_POINT('',(-1.8,14.1,4.5));
#14519=CARTESIAN_POINT('',(-1.8,14.35,1.4));
#14520=CARTESIAN_POINT('Origin',(1.8,13.7,4.5));
#14521=CARTESIAN_POINT('',(1.8,13.7,1.4));
#14522=CARTESIAN_POINT('',(1.8,13.7,4.5));
#14523=CARTESIAN_POINT('',(1.8,13.7,1.4));
#14524=CARTESIAN_POINT('',(1.8,14.1,1.4));
#14525=CARTESIAN_POINT('',(1.8,14.35,1.4));
#14526=CARTESIAN_POINT('',(1.8,14.1,4.5));
#14527=CARTESIAN_POINT('',(1.8,14.1,1.4));
#14528=CARTESIAN_POINT('',(1.8,13.7,4.5));
#14529=CARTESIAN_POINT('Origin',(-1.8,13.7,4.5));
#14530=CARTESIAN_POINT('',(1.8,13.7,4.5));
#14531=CARTESIAN_POINT('',(1.8,14.1,4.5));
#14532=CARTESIAN_POINT('Origin',(0.,14.1,2.95));
#14533=CARTESIAN_POINT('',(0.,14.1,1.4));
#14534=CARTESIAN_POINT('Origin',(0.,13.7,2.95));
#14535=CARTESIAN_POINT('',(0.,13.7,1.4));
#14536=CARTESIAN_POINT('Origin',(2.5,17.5,1.));
#14537=CARTESIAN_POINT('',(2.5,17.5,1.));
#14538=CARTESIAN_POINT('',(-2.5,17.5,1.));
#14539=CARTESIAN_POINT('',(2.5,17.5,1.));
#14540=CARTESIAN_POINT('',(-2.5,17.5,1.4));
#14541=CARTESIAN_POINT('',(-2.5,17.5,1.));
#14542=CARTESIAN_POINT('',(2.5,17.5,1.4));
#14543=CARTESIAN_POINT('',(2.5,17.5,1.4));
#14544=CARTESIAN_POINT('',(2.5,17.5,1.));
#14545=CARTESIAN_POINT('Origin',(2.5,12.5,1.));
#14546=CARTESIAN_POINT('',(2.5,12.5,1.));
#14547=CARTESIAN_POINT('',(2.5,12.5,1.));
#14548=CARTESIAN_POINT('',(2.5,12.5,1.4));
#14549=CARTESIAN_POINT('',(2.5,12.5,1.4));
#14550=CARTESIAN_POINT('',(2.5,12.5,1.));
#14551=CARTESIAN_POINT('Origin',(-2.5,12.5,1.));
#14552=CARTESIAN_POINT('',(-2.5,12.5,1.));
#14553=CARTESIAN_POINT('',(-2.5,12.5,1.));
#14554=CARTESIAN_POINT('',(-2.5,12.5,1.4));
#14555=CARTESIAN_POINT('',(-2.5,12.5,1.4));
#14556=CARTESIAN_POINT('',(-2.5,12.5,1.));
#14557=CARTESIAN_POINT('Origin',(-2.5,17.5,1.));
#14558=CARTESIAN_POINT('',(-2.5,17.5,1.));
#14559=CARTESIAN_POINT('',(-2.5,17.5,1.4));
#14560=CARTESIAN_POINT('Origin',(0.,15.,1.4));
#14561=CARTESIAN_POINT('Origin',(0.,15.,1.));
#16165=UNCERTAINTY_MEASURE_WITH_UNIT(LENGTH_MEASURE(0.001),#16282,
'DISTANCE_ACCURACY_VALUE',
'Maximum model space distance between geometric entities at asserted c
onnectivities');
#16212=UNCERTAINTY_MEASURE_WITH_UNIT(LENGTH_MEASURE(0.001),#16282,
'DISTANCE_ACCURACY_VALUE',
'Maximum model space distance between geometric entities at asserted c
onnectivities');
#16234=(
GEOMETRIC_REPRESENTATION_CONTEXT(3)
GLOBAL_UNCERTAINTY_ASSIGNED_CONTEXT((#16165))
GLOBAL_UNIT_ASSIGNED_CONTEXT((#16282,#16284,#16285))
REPRESENTATION_CONTEXT('','3D')
);
#16281=(
GEOMETRIC_REPRESENTATION_CONTEXT(3)
GLOBAL_UNCERTAINTY_ASSIGNED_CONTEXT((#16212))
GLOBAL_UNIT_ASSIGNED_CONTEXT((#16282,#16284,#16285))
REPRESENTATION_CONTEXT('','3D')
);
#16282=(
LENGTH_UNIT()
NAMED_UNIT(*)
SI_UNIT(.CENTI.,.METRE.)
);
#16284=(
NAMED_UNIT(*)
PLANE_ANGLE_UNIT()
SI_UNIT($,.RADIAN.)
);
#16285=(
NAMED_UNIT(*)
SI_UNIT($,.STERADIAN.)
SOLID_ANGLE_UNIT()
);
#16307=SHAPE_DEFINITION_REPRESENTATION(#16401,#16540);
#16401=PRODUCT_DEFINITION_SHAPE('',$,#16609);
#16540=SHAPE_REPRESENTATION('',(#9533),#16234);
#16587=PRODUCT_DEFINITION_CONTEXT('part definition',#16793,'design');
#16609=PRODUCT_DEFINITION('Roller bracket','Roller bracket',#16677,#16587);
#16677=PRODUCT_DEFINITION_FORMATION('',$,#16816);
#16793=APPLICATION_CONTEXT(
'Core Data for Automotive Mechanical Design Process');
#16794=PRODUCT_CONTEXT('part definition',#16793,'mechanical');
#16816=PRODUCT('Roller bracket','Roller bracket','Roller bracket',(#16794));
#16905=COLOUR_RGB('Dark Blue',0.08,0.2,0.34);
#16906=FILL_AREA_STYLE_COLOUR('',#16905);
#16907=FILL_AREA_STYLE('',(#16906));
#16908=SURFACE_STYLE_FILL_AREA(#16907);
#16909=SURFACE_SIDE_STYLE('',(#16908));
#16910=SURFACE_STYLE_USAGE(.BOTH.,#16909);
#16911=PRESENTATION_STYLE_ASSIGNMENT((#16910));
ENDSEC;
END-ISO-10303-21;
